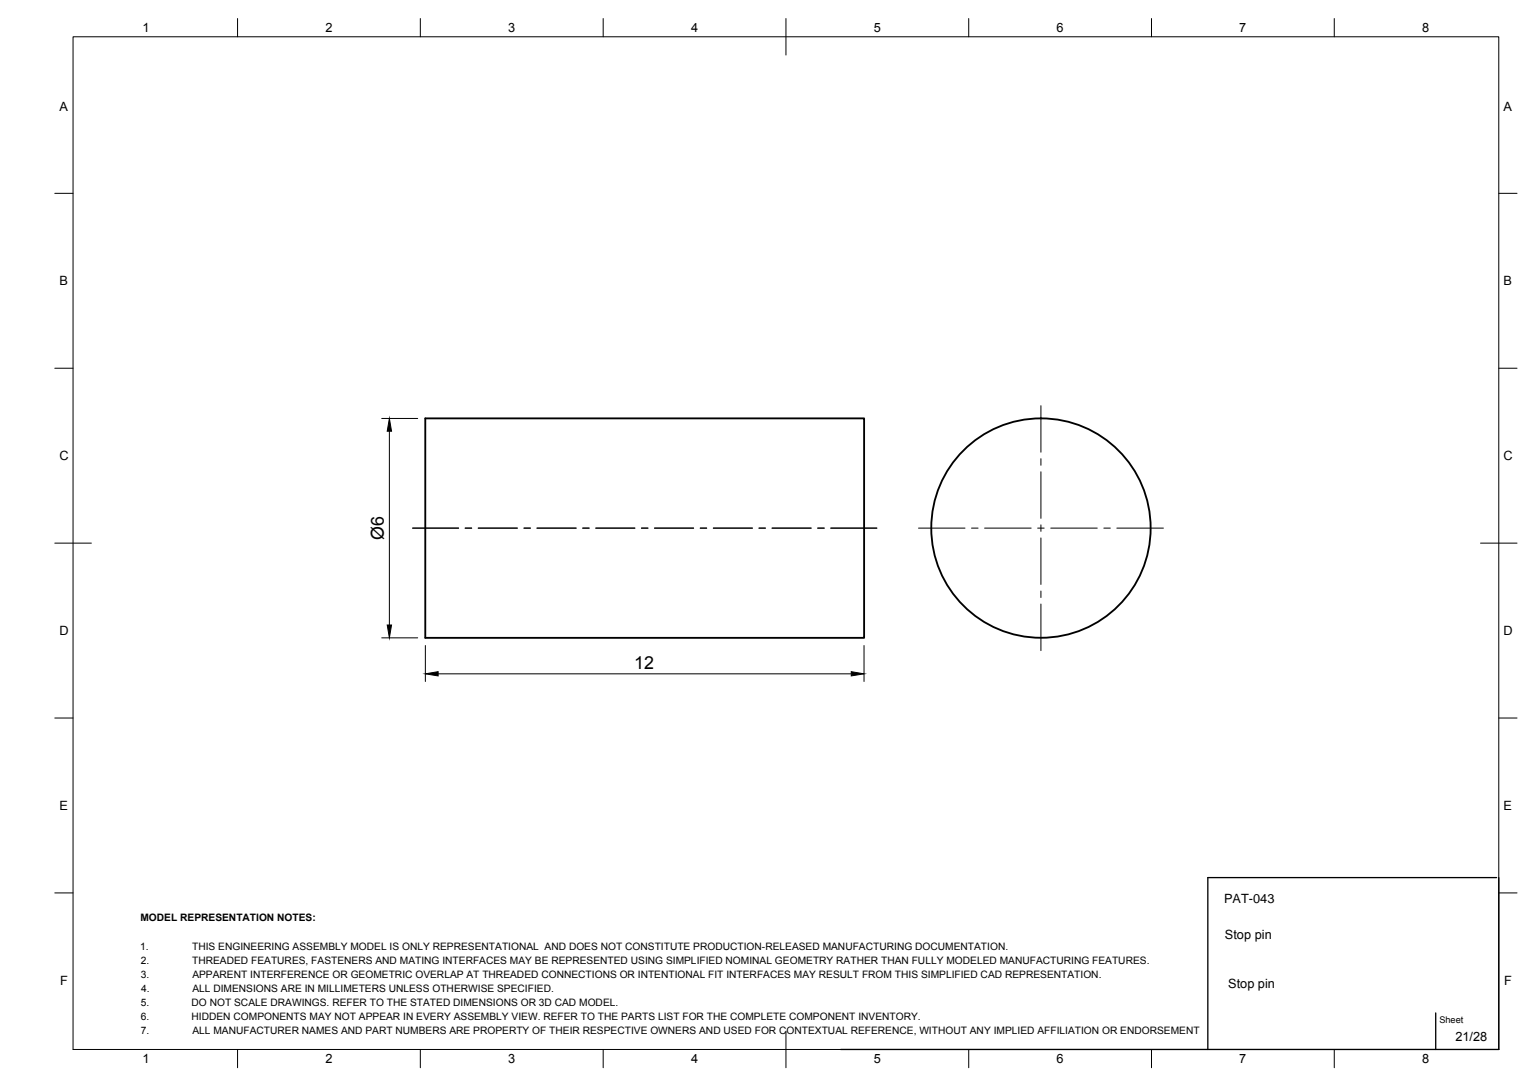
ISO-10303-21;
HEADER;
/* Generated by software containing ST-Developer
 * from STEP Tools, Inc. (www.steptools.com) 
 */

FILE_DESCRIPTION(
/* description */ ('Four-valve pipe header'),
/* implementation_level */ '2;1');

FILE_NAME(
/* name */ 'Stop pin.step',
/* time_stamp */ '2026-10-29T16:56:19-07:00',
/* author */ (''),
/* organization */ (''),
/* preprocessor_version */ 'ST-DEVELOPER v20.2',
/* originating_system */ 'Autodesk Translation Framework v15.17.0.0',
/* authorisation */ '');

FILE_SCHEMA (('AUTOMOTIVE_DESIGN { 1 0 10303 214 3 1 1 }'));
ENDSEC;

DATA;
#10=MECHANICAL_DESIGN_GEOMETRIC_PRESENTATION_REPRESENTATION('',(#352),#10119);
#300=SHAPE_REPRESENTATION_RELATIONSHIP('SRR','None',#10262,#326);
#326=ADVANCED_BREP_SHAPE_REPRESENTATION('',(#376),#10111);
#352=STYLED_ITEM('',(#10470),#376);
#376=MANIFOLD_SOLID_BREP('Body1',#5600);
#691=PLANE('',#6408);
#692=PLANE('',#6409);
#1011=FACE_OUTER_BOUND('',#1443,.T.);
#1012=FACE_OUTER_BOUND('',#1444,.T.);
#1013=FACE_OUTER_BOUND('',#1445,.T.);
#1443=EDGE_LOOP('',(#4873,#4874,#4875,#4876));
#1444=EDGE_LOOP('',(#4877));
#1445=EDGE_LOOP('',(#4878));
#1833=LINE('',#9704,#2251);
#2251=VECTOR('',#7906,0.3);
#2547=CIRCLE('',#6406,0.3);
#2548=CIRCLE('',#6407,0.3);
#2948=VERTEX_POINT('',#9701);
#2949=VERTEX_POINT('',#9703);
#3603=EDGE_CURVE('',#2948,#2948,#2547,.T.);
#3604=EDGE_CURVE('',#2948,#2949,#1833,.T.);
#3605=EDGE_CURVE('',#2949,#2949,#2548,.T.);
#4873=ORIENTED_EDGE('',*,*,#3603,.F.);
#4874=ORIENTED_EDGE('',*,*,#3604,.T.);
#4875=ORIENTED_EDGE('',*,*,#3605,.T.);
#4876=ORIENTED_EDGE('',*,*,#3604,.F.);
#4877=ORIENTED_EDGE('',*,*,#3603,.T.);
#4878=ORIENTED_EDGE('',*,*,#3605,.F.);
#5239=CYLINDRICAL_SURFACE('',#6405,0.3);
#5511=ADVANCED_FACE('',(#1011),#5239,.T.);
#5512=ADVANCED_FACE('',(#1012),#691,.T.);
#5513=ADVANCED_FACE('',(#1013),#692,.F.);
#5600=CLOSED_SHELL('',(#5511,#5512,#5513));
#6404=AXIS2_PLACEMENT_3D('',#9699,#7900,#7901);
#6405=AXIS2_PLACEMENT_3D('',#9700,#7902,#7903);
#6406=AXIS2_PLACEMENT_3D('',#9702,#7904,#7905);
#6407=AXIS2_PLACEMENT_3D('',#9705,#7907,#7908);
#6408=AXIS2_PLACEMENT_3D('',#9706,#7909,#7910);
#6409=AXIS2_PLACEMENT_3D('',#9707,#7911,#7912);
#7900=DIRECTION('axis',(0.,0.,1.));
#7901=DIRECTION('refdir',(1.,0.,0.));
#7902=DIRECTION('center_axis',(0.,0.,1.));
#7903=DIRECTION('ref_axis',(1.,0.,0.));
#7904=DIRECTION('center_axis',(0.,0.,1.));
#7905=DIRECTION('ref_axis',(1.,0.,0.));
#7906=DIRECTION('',(0.,0.,-1.));
#7907=DIRECTION('center_axis',(0.,0.,1.));
#7908=DIRECTION('ref_axis',(1.,0.,0.));
#7909=DIRECTION('center_axis',(0.,0.,1.));
#7910=DIRECTION('ref_axis',(1.,0.,0.));
#7911=DIRECTION('center_axis',(0.,0.,1.));
#7912=DIRECTION('ref_axis',(1.,0.,0.));
#9699=CARTESIAN_POINT('',(0.,0.,0.));
#9700=CARTESIAN_POINT('Origin',(3.,1.1,8.2));
#9701=CARTESIAN_POINT('',(2.7,1.1,9.4));
#9702=CARTESIAN_POINT('Origin',(3.,1.1,9.4));
#9703=CARTESIAN_POINT('',(2.7,1.1,8.2));
#9704=CARTESIAN_POINT('',(2.7,1.1,8.2));
#9705=CARTESIAN_POINT('Origin',(3.,1.1,8.2));
#9706=CARTESIAN_POINT('Origin',(3.,1.1,9.4));
#9707=CARTESIAN_POINT('Origin',(3.,1.1,8.2));
#10080=UNCERTAINTY_MEASURE_WITH_UNIT(LENGTH_MEASURE(0.001),#10120,
'DISTANCE_ACCURACY_VALUE',
'Maximum model space distance between geometric entities at asserted c
onnectivities');
#10088=UNCERTAINTY_MEASURE_WITH_UNIT(LENGTH_MEASURE(0.001),#10120,
'DISTANCE_ACCURACY_VALUE',
'Maximum model space distance between geometric entities at asserted c
onnectivities');
#10111=(
GEOMETRIC_REPRESENTATION_CONTEXT(3)
GLOBAL_UNCERTAINTY_ASSIGNED_CONTEXT((#10080))
GLOBAL_UNIT_ASSIGNED_CONTEXT((#10120,#10122,#10123))
REPRESENTATION_CONTEXT('','3D')
);
#10119=(
GEOMETRIC_REPRESENTATION_CONTEXT(3)
GLOBAL_UNCERTAINTY_ASSIGNED_CONTEXT((#10088))
GLOBAL_UNIT_ASSIGNED_CONTEXT((#10120,#10122,#10123))
REPRESENTATION_CONTEXT('','3D')
);
#10120=(
LENGTH_UNIT()
NAMED_UNIT(*)
SI_UNIT(.CENTI.,.METRE.)
);
#10122=(
NAMED_UNIT(*)
PLANE_ANGLE_UNIT()
SI_UNIT($,.RADIAN.)
);
#10123=(
NAMED_UNIT(*)
SI_UNIT($,.STERADIAN.)
SOLID_ANGLE_UNIT()
);
#10146=SHAPE_DEFINITION_REPRESENTATION(#10176,#10262);
#10176=PRODUCT_DEFINITION_SHAPE('',$,#10293);
#10262=SHAPE_REPRESENTATION('',(#6404),#10111);
#10270=PRODUCT_DEFINITION_CONTEXT('part definition',#10362,'design');
#10293=PRODUCT_DEFINITION('Stop pin','Stop pin',#10323,#10270);
#10323=PRODUCT_DEFINITION_FORMATION('',$,#10386);
#10362=APPLICATION_CONTEXT(
'Core Data for Automotive Mechanical Design Process');
#10363=PRODUCT_CONTEXT('part definition',#10362,'mechanical');
#10386=PRODUCT('Stop pin','Stop pin','Stop pin',(#10363));
#10464=COLOUR_RGB('Grey',0.48,0.52,0.57);
#10465=FILL_AREA_STYLE_COLOUR('',#10464);
#10466=FILL_AREA_STYLE('',(#10465));
#10467=SURFACE_STYLE_FILL_AREA(#10466);
#10468=SURFACE_SIDE_STYLE('',(#10467));
#10469=SURFACE_STYLE_USAGE(.BOTH.,#10468);
#10470=PRESENTATION_STYLE_ASSIGNMENT((#10469));
ENDSEC;
END-ISO-10303-21;
